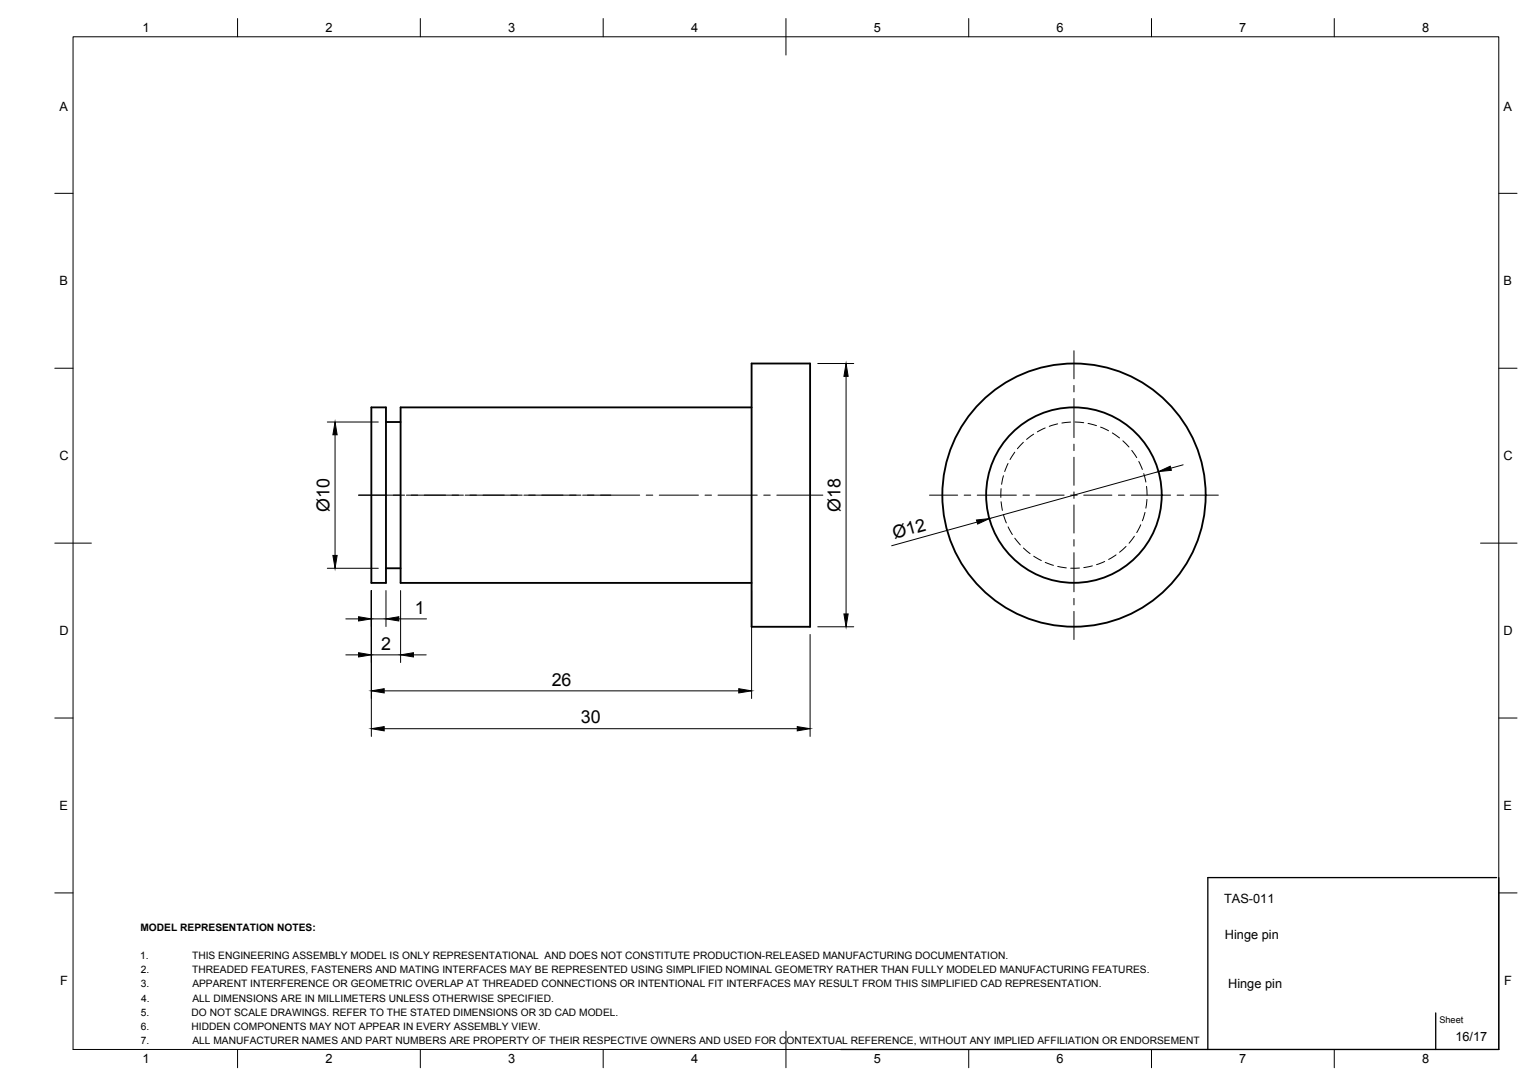
ISO-10303-21;
HEADER;
/* Generated by software containing ST-Developer
 * from STEP Tools, Inc. (www.steptools.com) 
 */

FILE_DESCRIPTION(
/* description */ (
'Independent manual bench leaf bending machine,200mm work width. Fabri
cated welded frame and folding leaf, repeated bushed and fully retaine
d hinge hardware, two handles with bonded grips, beveled clamping beam
 and modeledM12 clamp screws.2mm omitted-workpiece assembly reference 
gap, not a capacity claim. Native135deg hinge travel. Weld sizing, pro
duction fits, material condition, bending capacity, strength and life 
unassigned.'),
/* implementation_level */ '2;1');

FILE_NAME(
/* name */ 'Hinge pin.step',
/* time_stamp */ '2026-11-14T09:11:34-08:00',
/* author */ (''),
/* organization */ (''),
/* preprocessor_version */ 'ST-DEVELOPER v20.2',
/* originating_system */ 'Autodesk Translation Framework v15.17.0.0',
/* authorisation */ '');

FILE_SCHEMA (('AUTOMOTIVE_DESIGN { 1 0 10303 214 3 1 1 }'));
ENDSEC;

DATA;
#10=MECHANICAL_DESIGN_GEOMETRIC_PRESENTATION_REPRESENTATION('',(#461),#37701);
#425=SHAPE_REPRESENTATION_RELATIONSHIP('SRR','None',#37794,#443);
#443=ADVANCED_BREP_SHAPE_REPRESENTATION('',(#479),#37698);
#461=STYLED_ITEM('',(#37884),#479);
#479=MANIFOLD_SOLID_BREP('Body1',#4159);
#511=FACE_BOUND('',#1038,.T.);
#512=FACE_BOUND('',#1040,.T.);
#513=FACE_BOUND('',#1043,.T.);
#591=PLANE('',#4639);
#592=PLANE('',#4641);
#593=PLANE('',#4645);
#594=PLANE('',#4650);
#595=PLANE('',#4652);
#795=FACE_OUTER_BOUND('',#1036,.T.);
#796=FACE_OUTER_BOUND('',#1037,.T.);
#797=FACE_OUTER_BOUND('',#1039,.T.);
#798=FACE_OUTER_BOUND('',#1041,.T.);
#799=FACE_OUTER_BOUND('',#1042,.T.);
#800=FACE_OUTER_BOUND('',#1044,.T.);
#801=FACE_OUTER_BOUND('',#1045,.T.);
#802=FACE_OUTER_BOUND('',#1046,.T.);
#803=FACE_OUTER_BOUND('',#1047,.T.);
#1036=EDGE_LOOP('',(#3751,#3752,#3753,#3754));
#1037=EDGE_LOOP('',(#3755));
#1038=EDGE_LOOP('',(#3756));
#1039=EDGE_LOOP('',(#3757));
#1040=EDGE_LOOP('',(#3758));
#1041=EDGE_LOOP('',(#3759,#3760,#3761,#3762));
#1042=EDGE_LOOP('',(#3763));
#1043=EDGE_LOOP('',(#3764));
#1044=EDGE_LOOP('',(#3765,#3766,#3767,#3768));
#1045=EDGE_LOOP('',(#3769));
#1046=EDGE_LOOP('',(#3770,#3771,#3772,#3773));
#1047=EDGE_LOOP('',(#3774));
#1295=LINE('',#37561,#1544);
#1296=LINE('',#37572,#1545);
#1297=LINE('',#37580,#1546);
#1298=LINE('',#37584,#1547);
#1544=VECTOR('',#5496,5.);
#1545=VECTOR('',#5511,6.);
#1546=VECTOR('',#5520,9.);
#1547=VECTOR('',#5527,6.);
#1621=CIRCLE('',#4637,5.);
#1622=CIRCLE('',#4638,5.);
#1623=CIRCLE('',#4640,6.);
#1624=CIRCLE('',#4642,6.);
#1625=CIRCLE('',#4644,6.);
#1626=CIRCLE('',#4646,9.);
#1627=CIRCLE('',#4647,6.);
#1628=CIRCLE('',#4649,9.);
#2033=VERTEX_POINT('',#37558);
#2034=VERTEX_POINT('',#37560);
#2035=VERTEX_POINT('',#37564);
#2036=VERTEX_POINT('',#37567);
#2037=VERTEX_POINT('',#37570);
#2038=VERTEX_POINT('',#37574);
#2039=VERTEX_POINT('',#37576);
#2040=VERTEX_POINT('',#37579);
#2609=EDGE_CURVE('',#2033,#2033,#1621,.T.);
#2610=EDGE_CURVE('',#2033,#2034,#1295,.T.);
#2611=EDGE_CURVE('',#2034,#2034,#1622,.T.);
#2612=EDGE_CURVE('',#2035,#2035,#1623,.T.);
#2613=EDGE_CURVE('',#2036,#2036,#1624,.T.);
#2614=EDGE_CURVE('',#2037,#2037,#1625,.T.);
#2615=EDGE_CURVE('',#2037,#2036,#1296,.T.);
#2616=EDGE_CURVE('',#2038,#2038,#1626,.T.);
#2617=EDGE_CURVE('',#2039,#2039,#1627,.T.);
#2618=EDGE_CURVE('',#2038,#2040,#1297,.T.);
#2619=EDGE_CURVE('',#2040,#2040,#1628,.T.);
#2620=EDGE_CURVE('',#2035,#2039,#1298,.T.);
#3751=ORIENTED_EDGE('',*,*,#2609,.F.);
#3752=ORIENTED_EDGE('',*,*,#2610,.T.);
#3753=ORIENTED_EDGE('',*,*,#2611,.T.);
#3754=ORIENTED_EDGE('',*,*,#2610,.F.);
#3755=ORIENTED_EDGE('',*,*,#2612,.F.);
#3756=ORIENTED_EDGE('',*,*,#2611,.F.);
#3757=ORIENTED_EDGE('',*,*,#2613,.F.);
#3758=ORIENTED_EDGE('',*,*,#2609,.T.);
#3759=ORIENTED_EDGE('',*,*,#2614,.F.);
#3760=ORIENTED_EDGE('',*,*,#2615,.T.);
#3761=ORIENTED_EDGE('',*,*,#2613,.T.);
#3762=ORIENTED_EDGE('',*,*,#2615,.F.);
#3763=ORIENTED_EDGE('',*,*,#2616,.T.);
#3764=ORIENTED_EDGE('',*,*,#2617,.F.);
#3765=ORIENTED_EDGE('',*,*,#2616,.F.);
#3766=ORIENTED_EDGE('',*,*,#2618,.T.);
#3767=ORIENTED_EDGE('',*,*,#2619,.T.);
#3768=ORIENTED_EDGE('',*,*,#2618,.F.);
#3769=ORIENTED_EDGE('',*,*,#2619,.F.);
#3770=ORIENTED_EDGE('',*,*,#2612,.T.);
#3771=ORIENTED_EDGE('',*,*,#2620,.T.);
#3772=ORIENTED_EDGE('',*,*,#2617,.T.);
#3773=ORIENTED_EDGE('',*,*,#2620,.F.);
#3774=ORIENTED_EDGE('',*,*,#2614,.T.);
#3924=CYLINDRICAL_SURFACE('',#4636,5.);
#3925=CYLINDRICAL_SURFACE('',#4643,6.);
#3926=CYLINDRICAL_SURFACE('',#4648,9.);
#3927=CYLINDRICAL_SURFACE('',#4651,6.);
#4125=ADVANCED_FACE('',(#795),#3924,.T.);
#4126=ADVANCED_FACE('',(#796,#511),#591,.F.);
#4127=ADVANCED_FACE('',(#797,#512),#592,.F.);
#4128=ADVANCED_FACE('',(#798),#3925,.T.);
#4129=ADVANCED_FACE('',(#799,#513),#593,.T.);
#4130=ADVANCED_FACE('',(#800),#3926,.T.);
#4131=ADVANCED_FACE('',(#801),#594,.F.);
#4132=ADVANCED_FACE('',(#802),#3927,.T.);
#4133=ADVANCED_FACE('',(#803),#595,.T.);
#4159=CLOSED_SHELL('',(#4125,#4126,#4127,#4128,#4129,#4130,#4131,#4132,
#4133));
#4635=AXIS2_PLACEMENT_3D('',#37556,#5490,#5491);
#4636=AXIS2_PLACEMENT_3D('',#37557,#5492,#5493);
#4637=AXIS2_PLACEMENT_3D('',#37559,#5494,#5495);
#4638=AXIS2_PLACEMENT_3D('',#37562,#5497,#5498);
#4639=AXIS2_PLACEMENT_3D('',#37563,#5499,#5500);
#4640=AXIS2_PLACEMENT_3D('',#37565,#5501,#5502);
#4641=AXIS2_PLACEMENT_3D('',#37566,#5503,#5504);
#4642=AXIS2_PLACEMENT_3D('',#37568,#5505,#5506);
#4643=AXIS2_PLACEMENT_3D('',#37569,#5507,#5508);
#4644=AXIS2_PLACEMENT_3D('',#37571,#5509,#5510);
#4645=AXIS2_PLACEMENT_3D('',#37573,#5512,#5513);
#4646=AXIS2_PLACEMENT_3D('',#37575,#5514,#5515);
#4647=AXIS2_PLACEMENT_3D('',#37577,#5516,#5517);
#4648=AXIS2_PLACEMENT_3D('',#37578,#5518,#5519);
#4649=AXIS2_PLACEMENT_3D('',#37581,#5521,#5522);
#4650=AXIS2_PLACEMENT_3D('',#37582,#5523,#5524);
#4651=AXIS2_PLACEMENT_3D('',#37583,#5525,#5526);
#4652=AXIS2_PLACEMENT_3D('',#37585,#5528,#5529);
#5490=DIRECTION('axis',(0.,0.,1.));
#5491=DIRECTION('refdir',(1.,0.,0.));
#5492=DIRECTION('center_axis',(0.,0.,1.));
#5493=DIRECTION('ref_axis',(1.,0.,0.));
#5494=DIRECTION('center_axis',(0.,0.,1.));
#5495=DIRECTION('ref_axis',(1.,0.,0.));
#5496=DIRECTION('',(0.,0.,-1.));
#5497=DIRECTION('center_axis',(0.,0.,1.));
#5498=DIRECTION('ref_axis',(1.,0.,0.));
#5499=DIRECTION('center_axis',(0.,0.,-1.));
#5500=DIRECTION('ref_axis',(-1.,0.,0.));
#5501=DIRECTION('center_axis',(0.,0.,-1.));
#5502=DIRECTION('ref_axis',(1.,0.,0.));
#5503=DIRECTION('center_axis',(0.,0.,1.));
#5504=DIRECTION('ref_axis',(1.,0.,0.));
#5505=DIRECTION('center_axis',(0.,0.,1.));
#5506=DIRECTION('ref_axis',(1.,0.,0.));
#5507=DIRECTION('center_axis',(0.,0.,1.));
#5508=DIRECTION('ref_axis',(1.,0.,0.));
#5509=DIRECTION('center_axis',(0.,0.,1.));
#5510=DIRECTION('ref_axis',(1.,0.,0.));
#5511=DIRECTION('',(0.,0.,-1.));
#5512=DIRECTION('center_axis',(0.,0.,1.));
#5513=DIRECTION('ref_axis',(1.,0.,0.));
#5514=DIRECTION('center_axis',(0.,0.,1.));
#5515=DIRECTION('ref_axis',(1.,0.,0.));
#5516=DIRECTION('center_axis',(0.,0.,1.));
#5517=DIRECTION('ref_axis',(1.,0.,0.));
#5518=DIRECTION('center_axis',(0.,0.,1.));
#5519=DIRECTION('ref_axis',(1.,0.,0.));
#5520=DIRECTION('',(0.,0.,-1.));
#5521=DIRECTION('center_axis',(0.,0.,1.));
#5522=DIRECTION('ref_axis',(1.,0.,0.));
#5523=DIRECTION('center_axis',(0.,0.,1.));
#5524=DIRECTION('ref_axis',(1.,0.,0.));
#5525=DIRECTION('center_axis',(0.,0.,1.));
#5526=DIRECTION('ref_axis',(1.,0.,0.));
#5527=DIRECTION('',(0.,0.,-1.));
#5528=DIRECTION('center_axis',(0.,0.,1.));
#5529=DIRECTION('ref_axis',(1.,0.,0.));
#37556=CARTESIAN_POINT('',(0.,0.,0.));
#37557=CARTESIAN_POINT('Origin',(0.,0.,24.5));
#37558=CARTESIAN_POINT('',(-5.,-6.12323399573677E-16,25.));
#37559=CARTESIAN_POINT('Origin',(0.,0.,25.));
#37560=CARTESIAN_POINT('',(-5.,-6.12323399573677E-16,24.));
#37561=CARTESIAN_POINT('',(-5.,-6.12323399573677E-16,24.5));
#37562=CARTESIAN_POINT('Origin',(0.,0.,24.));
#37563=CARTESIAN_POINT('Origin',(9.,0.,24.));
#37564=CARTESIAN_POINT('',(-6.,7.34788079488412E-16,24.));
#37565=CARTESIAN_POINT('Origin',(0.,0.,24.));
#37566=CARTESIAN_POINT('Origin',(5.,0.,25.));
#37567=CARTESIAN_POINT('',(-6.,-7.34788079488412E-16,25.));
#37568=CARTESIAN_POINT('Origin',(0.,0.,25.));
#37569=CARTESIAN_POINT('Origin',(0.,0.,0.));
#37570=CARTESIAN_POINT('',(-6.,-7.34788079488412E-16,26.));
#37571=CARTESIAN_POINT('Origin',(0.,0.,26.));
#37572=CARTESIAN_POINT('',(-6.,-7.34788079488412E-16,0.));
#37573=CARTESIAN_POINT('Origin',(0.,0.,0.));
#37574=CARTESIAN_POINT('',(-9.,-1.10218211923262E-15,0.));
#37575=CARTESIAN_POINT('Origin',(0.,0.,0.));
#37576=CARTESIAN_POINT('',(-6.,-7.34788079488412E-16,0.));
#37577=CARTESIAN_POINT('Origin',(0.,0.,0.));
#37578=CARTESIAN_POINT('Origin',(0.,0.,-4.));
#37579=CARTESIAN_POINT('',(-9.,-1.10218211923262E-15,-4.));
#37580=CARTESIAN_POINT('',(-9.,-1.10218211923262E-15,-4.));
#37581=CARTESIAN_POINT('Origin',(0.,0.,-4.));
#37582=CARTESIAN_POINT('Origin',(0.,0.,-4.));
#37583=CARTESIAN_POINT('Origin',(0.,0.,0.));
#37584=CARTESIAN_POINT('',(-6.,-7.34788079488412E-16,0.));
#37585=CARTESIAN_POINT('Origin',(0.,0.,26.));
#37678=UNCERTAINTY_MEASURE_WITH_UNIT(LENGTH_MEASURE(0.01),#37702,
'DISTANCE_ACCURACY_VALUE',
'Maximum model space distance between geometric entities at asserted c
onnectivities');
#37681=UNCERTAINTY_MEASURE_WITH_UNIT(LENGTH_MEASURE(0.01),#37702,
'DISTANCE_ACCURACY_VALUE',
'Maximum model space distance between geometric entities at asserted c
onnectivities');
#37698=(
GEOMETRIC_REPRESENTATION_CONTEXT(3)
GLOBAL_UNCERTAINTY_ASSIGNED_CONTEXT((#37678))
GLOBAL_UNIT_ASSIGNED_CONTEXT((#37702,#37704,#37705))
REPRESENTATION_CONTEXT('','3D')
);
#37701=(
GEOMETRIC_REPRESENTATION_CONTEXT(3)
GLOBAL_UNCERTAINTY_ASSIGNED_CONTEXT((#37681))
GLOBAL_UNIT_ASSIGNED_CONTEXT((#37702,#37704,#37705))
REPRESENTATION_CONTEXT('','3D')
);
#37702=(
LENGTH_UNIT()
NAMED_UNIT(*)
SI_UNIT(.MILLI.,.METRE.)
);
#37704=(
NAMED_UNIT(*)
PLANE_ANGLE_UNIT()
SI_UNIT($,.RADIAN.)
);
#37705=(
NAMED_UNIT(*)
SI_UNIT($,.STERADIAN.)
SOLID_ANGLE_UNIT()
);
#37722=SHAPE_DEFINITION_REPRESENTATION(#37741,#37794);
#37741=PRODUCT_DEFINITION_SHAPE('',$,#37814);
#37794=SHAPE_REPRESENTATION('',(#4635),#37698);
#37797=PRODUCT_DEFINITION_CONTEXT('part definition',#37856,'design');
#37814=PRODUCT_DEFINITION('Hinge pin','Hinge pin',#37833,#37797);
#37833=PRODUCT_DEFINITION_FORMATION('',$,#37874);
#37856=APPLICATION_CONTEXT(
'Core Data for Automotive Mechanical Design Process');
#37857=PRODUCT_CONTEXT('part definition',#37856,'mechanical');
#37874=PRODUCT('Hinge pin','Hinge pin','Hinge pin',(#37857));
#37884=PRESENTATION_STYLE_ASSIGNMENT((#37892));
#37892=SURFACE_STYLE_USAGE(.BOTH.,#37900);
#37900=SURFACE_SIDE_STYLE('',(#37908));
#37908=SURFACE_STYLE_FILL_AREA(#37916);
#37916=FILL_AREA_STYLE('Opaque(147,157,170)',(#37924));
#37924=FILL_AREA_STYLE_COLOUR('Opaque(147,157,170)',#37932);
#37932=COLOUR_RGB('Opaque(147,157,170)',0.576470588235294,0.615686274509804,
0.666666666666667);
ENDSEC;
END-ISO-10303-21;
